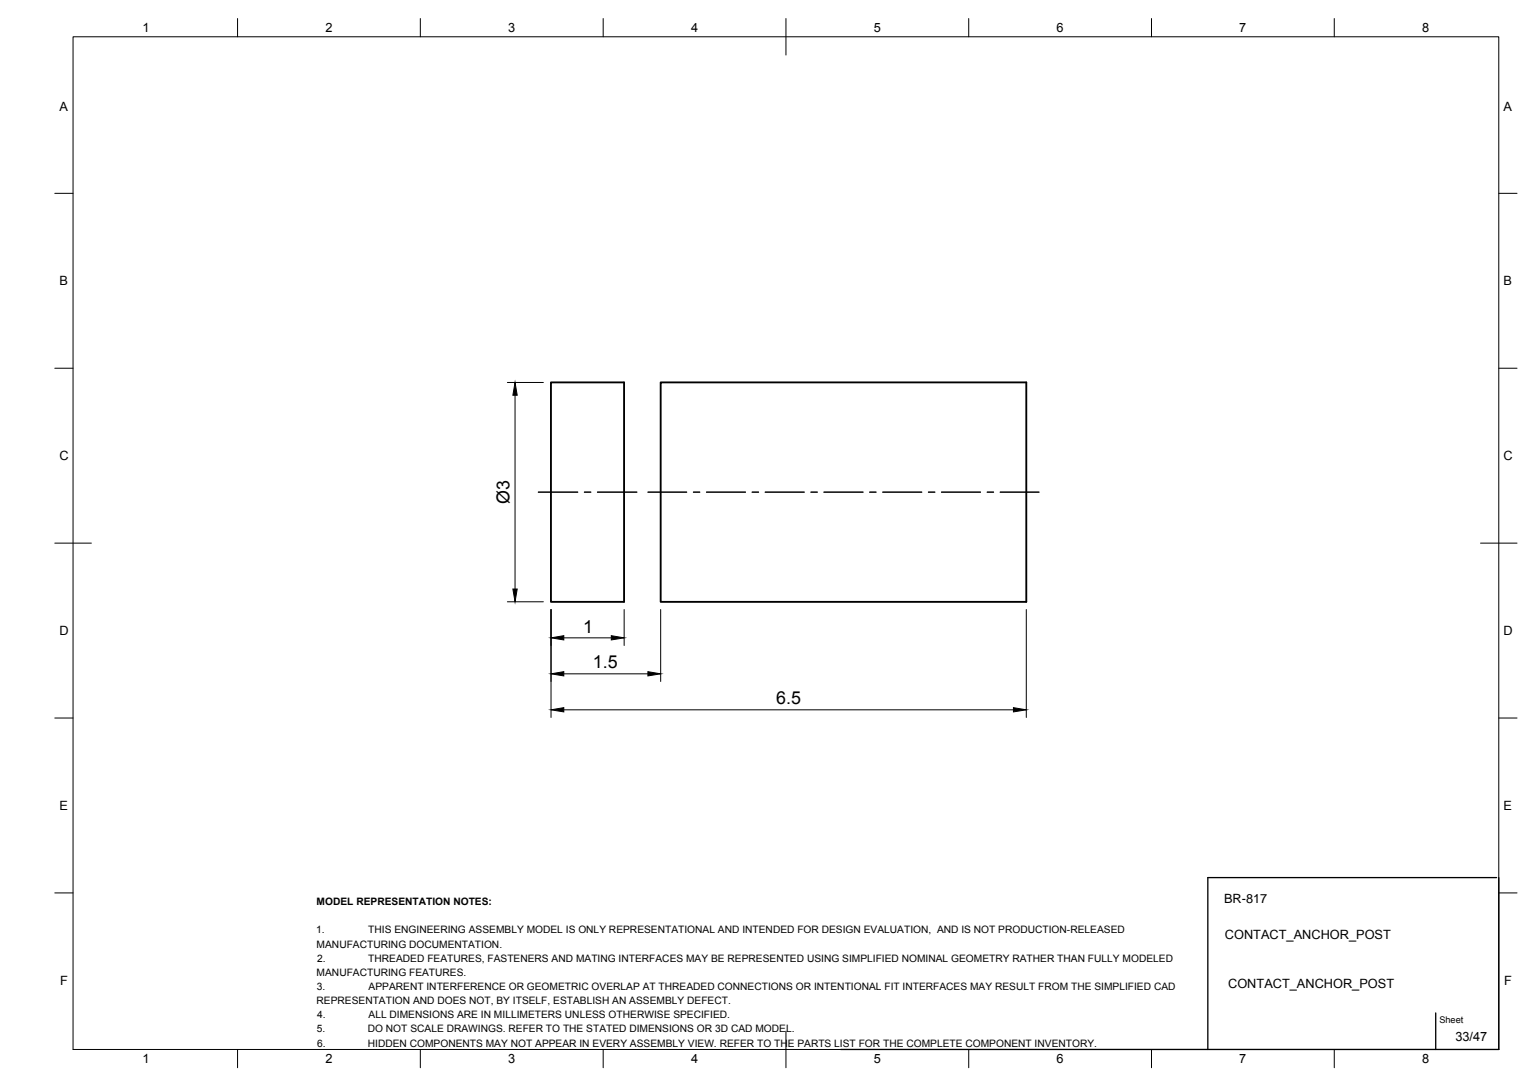
ISO-10303-21;
HEADER;
FILE_DESCRIPTION((''),'2;1');
FILE_NAME('CONTACT_ANCHOR_POST.step','2026-10-01T22:07:29-07:00',(''),(''),'','','');
FILE_SCHEMA (('AUTOMOTIVE_DESIGN { 1 0 10303 214 3 1 1 }'));
ENDSEC;
DATA;
#10=MECHANICAL_DESIGN_GEOMETRIC_PRESENTATION_REPRESENTATION('',(#565,#566),#15484);
#495=SHAPE_REPRESENTATION_RELATIONSHIP('SRR','None',#15645,#530) ;
#530=ADVANCED_BREP_SHAPE_REPRESENTATION('',(#606,#607),#15469) ;
#565=STYLED_ITEM('',(#15834),#606) ;
#566=STYLED_ITEM('',(#15834),#607) ;
#606=MANIFOLD_SOLID_BREP('CONTACT_ANCHOR_POST',#8276) ;
#607=MANIFOLD_SOLID_BREP('CONTACT_ANCHOR_POST',#8277) ;
#757=CYLINDRICAL_SURFACE('',#9526,0.15) ;
#758=CYLINDRICAL_SURFACE('',#9531,0.15) ;
#1221=CIRCLE('',#9527,0.15) ;
#1222=CIRCLE('',#9528,0.15) ;
#1223=CIRCLE('',#9532,0.15) ;
#1224=CIRCLE('',#9533,0.15) ;
#1712=FACE_OUTER_BOUND('',#2278,.T.) ;
#1713=FACE_OUTER_BOUND('',#2279,.T.) ;
#1714=FACE_OUTER_BOUND('',#2280,.T.) ;
#1715=FACE_OUTER_BOUND('',#2281,.T.) ;
#1716=FACE_OUTER_BOUND('',#2282,.T.) ;
#1717=FACE_OUTER_BOUND('',#2283,.T.) ;
#2278=EDGE_LOOP('',(#6873,#6874,#6875,#6876)) ;
#2279=EDGE_LOOP('',(#6877)) ;
#2280=EDGE_LOOP('',(#6878)) ;
#2281=EDGE_LOOP('',(#6879,#6880,#6881,#6882)) ;
#2282=EDGE_LOOP('',(#6883)) ;
#2283=EDGE_LOOP('',(#6884)) ;
#2784=LINE('',#14654,#3258) ;
#2785=LINE('',#14662,#3259) ;
#3258=VECTOR('',#11961,0.15) ;
#3259=VECTOR('',#11972,0.15) ;
#3921=VERTEX_POINT('',#14651) ;
#3922=VERTEX_POINT('',#14653) ;
#3923=VERTEX_POINT('',#14659) ;
#3924=VERTEX_POINT('',#14661) ;
#4941=EDGE_CURVE('',#3921,#3921,#1221,.T.) ;
#4942=EDGE_CURVE('',#3921,#3922,#2784,.T.) ;
#4943=EDGE_CURVE('',#3922,#3922,#1222,.T.) ;
#4944=EDGE_CURVE('',#3923,#3923,#1223,.T.) ;
#4945=EDGE_CURVE('',#3923,#3924,#2785,.T.) ;
#4946=EDGE_CURVE('',#3924,#3924,#1224,.T.) ;
#6873=ORIENTED_EDGE('',*,*,#4941,.F.) ;
#6874=ORIENTED_EDGE('',*,*,#4942,.T.) ;
#6875=ORIENTED_EDGE('',*,*,#4943,.F.) ;
#6876=ORIENTED_EDGE('',*,*,#4942,.F.) ;
#6877=ORIENTED_EDGE('',*,*,#4943,.T.) ;
#6878=ORIENTED_EDGE('',*,*,#4941,.T.) ;
#6879=ORIENTED_EDGE('',*,*,#4944,.F.) ;
#6880=ORIENTED_EDGE('',*,*,#4945,.T.) ;
#6881=ORIENTED_EDGE('',*,*,#4946,.F.) ;
#6882=ORIENTED_EDGE('',*,*,#4945,.F.) ;
#6883=ORIENTED_EDGE('',*,*,#4946,.T.) ;
#6884=ORIENTED_EDGE('',*,*,#4944,.T.) ;
#7685=PLANE('',#9529) ;
#7686=PLANE('',#9530) ;
#7687=PLANE('',#9534) ;
#7688=PLANE('',#9535) ;
#8099=ADVANCED_FACE('',(#1712),#757,.T.) ;
#8100=ADVANCED_FACE('',(#1713),#7685,.T.) ;
#8101=ADVANCED_FACE('',(#1714),#7686,.T.) ;
#8102=ADVANCED_FACE('',(#1715),#758,.T.) ;
#8103=ADVANCED_FACE('',(#1716),#7687,.T.) ;
#8104=ADVANCED_FACE('',(#1717),#7688,.T.) ;
#8276=CLOSED_SHELL('',(#8099,#8100,#8101)) ;
#8277=CLOSED_SHELL('',(#8102,#8103,#8104)) ;
#9525=AXIS2_PLACEMENT_3D('',#14649,#11955,#11956) ;
#9526=AXIS2_PLACEMENT_3D('',#14650,#11957,#11958) ;
#9527=AXIS2_PLACEMENT_3D('',#14652,#11959,#11960) ;
#9528=AXIS2_PLACEMENT_3D('',#14655,#11962,#11963) ;
#9529=AXIS2_PLACEMENT_3D('',#14656,#11964,#11965) ;
#9530=AXIS2_PLACEMENT_3D('',#14657,#11966,#11967) ;
#9531=AXIS2_PLACEMENT_3D('',#14658,#11968,#11969) ;
#9532=AXIS2_PLACEMENT_3D('',#14660,#11970,#11971) ;
#9533=AXIS2_PLACEMENT_3D('',#14663,#11973,#11974) ;
#9534=AXIS2_PLACEMENT_3D('',#14664,#11975,#11976) ;
#9535=AXIS2_PLACEMENT_3D('',#14665,#11977,#11978) ;
#11955=DIRECTION('axis',(0.,0.,1.)) ;
#11956=DIRECTION('refdir',(1.,0.,0.)) ;
#11957=DIRECTION('center_axis',(0.,0.,1.)) ;
#11958=DIRECTION('ref_axis',(1.,0.,0.)) ;
#11959=DIRECTION('center_axis',(0.,0.,1.)) ;
#11960=DIRECTION('ref_axis',(1.,0.,0.)) ;
#11961=DIRECTION('',(0.,0.,-1.)) ;
#11962=DIRECTION('center_axis',(0.,0.,-1.)) ;
#11963=DIRECTION('ref_axis',(1.,0.,0.)) ;
#11964=DIRECTION('center_axis',(0.,0.,-1.)) ;
#11965=DIRECTION('ref_axis',(-1.,0.,0.)) ;
#11966=DIRECTION('center_axis',(0.,0.,1.)) ;
#11967=DIRECTION('ref_axis',(1.,0.,0.)) ;
#11968=DIRECTION('center_axis',(0.,0.,1.)) ;
#11969=DIRECTION('ref_axis',(1.,0.,0.)) ;
#11970=DIRECTION('center_axis',(0.,0.,1.)) ;
#11971=DIRECTION('ref_axis',(1.,0.,0.)) ;
#11972=DIRECTION('',(0.,0.,-1.)) ;
#11973=DIRECTION('center_axis',(0.,0.,-1.)) ;
#11974=DIRECTION('ref_axis',(1.,0.,0.)) ;
#11975=DIRECTION('center_axis',(0.,0.,-1.)) ;
#11976=DIRECTION('ref_axis',(-1.,0.,0.)) ;
#11977=DIRECTION('center_axis',(0.,0.,1.)) ;
#11978=DIRECTION('ref_axis',(1.,0.,0.)) ;
#14649=CARTESIAN_POINT('',(0.,0.,0.)) ;
#14650=CARTESIAN_POINT('Origin',(-2.6,-1.75,0.55)) ;
#14651=CARTESIAN_POINT('',(-2.75,-1.75,0.8)) ;
#14652=CARTESIAN_POINT('Origin',(-2.6,-1.75,0.8)) ;
#14653=CARTESIAN_POINT('',(-2.75,-1.75,0.3)) ;
#14654=CARTESIAN_POINT('',(-2.75,-1.75,0.55)) ;
#14655=CARTESIAN_POINT('Origin',(-2.6,-1.75,0.3)) ;
#14656=CARTESIAN_POINT('Origin',(-2.6,-1.75,0.3)) ;
#14657=CARTESIAN_POINT('Origin',(-2.6,-1.75,0.8)) ;
#14658=CARTESIAN_POINT('Origin',(-2.6,-1.75,0.9)) ;
#14659=CARTESIAN_POINT('',(-2.75,-1.75,0.95)) ;
#14660=CARTESIAN_POINT('Origin',(-2.6,-1.75,0.95)) ;
#14661=CARTESIAN_POINT('',(-2.75,-1.75,0.85)) ;
#14662=CARTESIAN_POINT('',(-2.75,-1.75,0.9)) ;
#14663=CARTESIAN_POINT('Origin',(-2.6,-1.75,0.85)) ;
#14664=CARTESIAN_POINT('Origin',(-2.6,-1.75,0.85)) ;
#14665=CARTESIAN_POINT('Origin',(-2.6,-1.75,0.95)) ;
#15426=UNCERTAINTY_MEASURE_WITH_UNIT(LENGTH_MEASURE(0.001),#15485,
'DISTANCE_ACCURACY_VALUE',
'Maximum model space distance between geometric entities at asserted c
onnectivities') ;
#15441=UNCERTAINTY_MEASURE_WITH_UNIT(LENGTH_MEASURE(0.001),#15485,
'DISTANCE_ACCURACY_VALUE',
'Maximum model space distance between geometric entities at asserted c
onnectivities') ;
#15469=(
GEOMETRIC_REPRESENTATION_CONTEXT(3)
GLOBAL_UNCERTAINTY_ASSIGNED_CONTEXT((#15426))
GLOBAL_UNIT_ASSIGNED_CONTEXT((#15485,#15487,#15488))
REPRESENTATION_CONTEXT('','3D')
) ;
#15484=(
GEOMETRIC_REPRESENTATION_CONTEXT(3)
GLOBAL_UNCERTAINTY_ASSIGNED_CONTEXT((#15441))
GLOBAL_UNIT_ASSIGNED_CONTEXT((#15485,#15487,#15488))
REPRESENTATION_CONTEXT('','3D')
) ;
#15485=(
LENGTH_UNIT()
NAMED_UNIT(*)
SI_UNIT(.CENTI.,.METRE.)
) ;
#15487=(
NAMED_UNIT(*)
PLANE_ANGLE_UNIT()
SI_UNIT($,.RADIAN.)
) ;
#15488=(
NAMED_UNIT(*)
SI_UNIT($,.STERADIAN.)
SOLID_ANGLE_UNIT()
) ;
#15516=SHAPE_DEFINITION_REPRESENTATION(#15573,#15645) ;
#15573=PRODUCT_DEFINITION_SHAPE('',$,#15688) ;
#15645=SHAPE_REPRESENTATION('',(#9525),#15469) ;
#15660=PRODUCT_DEFINITION_CONTEXT('part definition',#15788,'design') ;
#15688=PRODUCT_DEFINITION('CONTACT_ANCHOR_POST',
'CONTACT_ANCHOR_POST',#15730,#15660) ;
#15730=PRODUCT_DEFINITION_FORMATION('',$,#15817) ;
#15788=APPLICATION_CONTEXT(
'Core Data for Automotive Mechanical Design Process') ;
#15789=PRODUCT_CONTEXT('part definition',#15788,'mechanical') ;
#15817=PRODUCT('CONTACT_ANCHOR_POST','CONTACT_ANCHOR_POST',$,(#15789)) ;
#15834=PRESENTATION_STYLE_ASSIGNMENT((#15846)) ;
#15846=SURFACE_STYLE_USAGE(.BOTH.,#15858) ;
#15858=SURFACE_SIDE_STYLE('',(#15870)) ;
#15870=SURFACE_STYLE_FILL_AREA(#15882) ;
#15882=FILL_AREA_STYLE('Brass - Polished',(#15894)) ;
#15894=FILL_AREA_STYLE_COLOUR('Brass - Polished',#15906) ;
#15906=COLOUR_RGB('Brass - Polished', 0.08235294, 0.09019608, 0.10196078) ;
ENDSEC;
END-ISO-10303-21;
